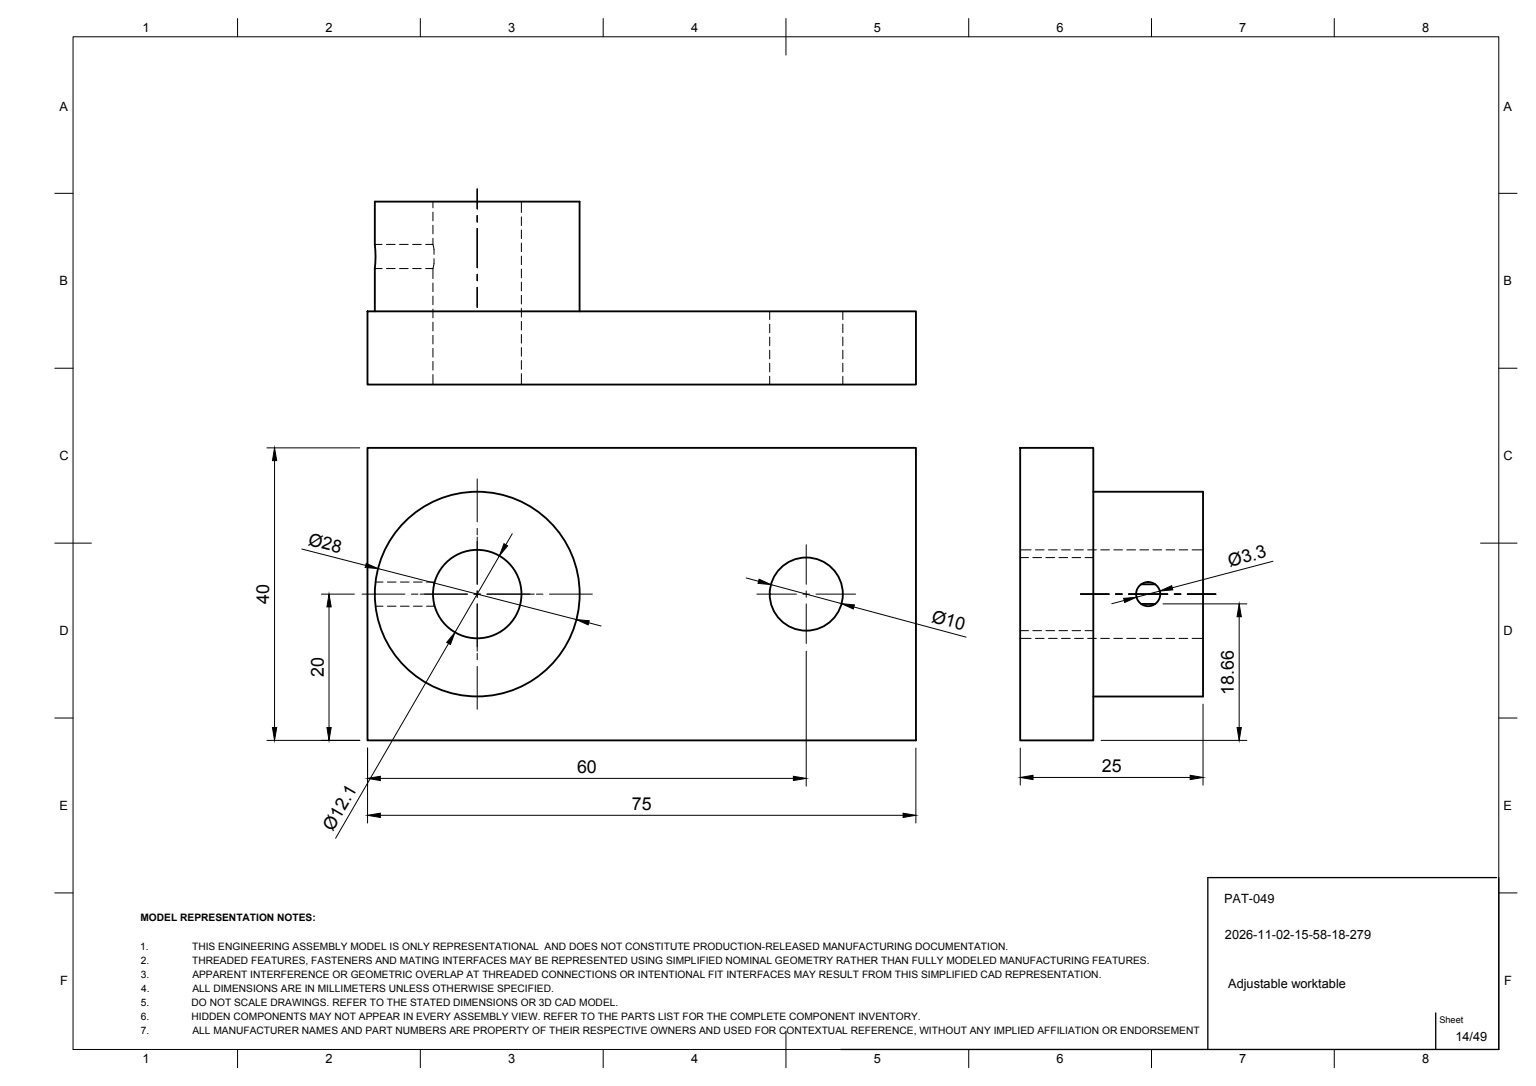
ISO-10303-21;
HEADER;
/* Generated by software containing ST-Developer
 * from STEP Tools, Inc. (www.steptools.com) 
 */

FILE_DESCRIPTION(
/* description */ ('Hand drill press frame (manual)'),
/* implementation_level */ '2;1');

FILE_NAME(
/* name */ 'Adjustable worktable.step',
/* time_stamp */ '2026-10-28T03:25:28-07:00',
/* author */ (''),
/* organization */ (''),
/* preprocessor_version */ 'ST-DEVELOPER v20.2',
/* originating_system */ 'Autodesk Translation Framework v15.17.0.0',
/* authorisation */ '');

FILE_SCHEMA (('AUTOMOTIVE_DESIGN { 1 0 10303 214 3 1 1 }'));
ENDSEC;

DATA;
#10=MECHANICAL_DESIGN_GEOMETRIC_PRESENTATION_REPRESENTATION('',(#628),#33299);
#501=B_SPLINE_CURVE_WITH_KNOTS('',3,(#18696,#18697,#18698,#18699,#18700,
#18701,#18702,#18703,#18704,#18705,#18706,#18707,#18708,#18709),
 .UNSPECIFIED.,.F.,.F.,(4,2,2,2,2,2,4),(0.598759573717651,0.624973342427791,
0.687463163426144,0.749952984424497,0.812442805422849,0.874932626421202,
0.901146395131343),.UNSPECIFIED.);
#502=B_SPLINE_CURVE_WITH_KNOTS('',3,(#18713,#18714,#18715,#18716,#18717,
#18718,#18719,#18720),.UNSPECIFIED.,.F.,.F.,(4,2,2,4),(0.249984328141499,
0.312474149139851,0.374963970138204,0.401177738848344),.UNSPECIFIED.);
#503=B_SPLINE_CURVE_WITH_KNOTS('',3,(#18724,#18725,#18726,#18727,#18728,
#18729,#18730,#18731,#18732,#18733,#18734,#18735,#18736,#18737,#18738,#18739,
#18740,#18741,#18742,#18743,#18744,#18745,#18746,#18747,#18748,#18749),
 .UNSPECIFIED.,.F.,.F.,(4,2,2,2,2,2,2,2,2,2,2,2,4),(0.,0.0622156192199746,
0.124431238439949,0.186646447577113,0.248861656714278,0.311076865851442,
0.373292074988606,0.43550769420858,0.497723313428555,0.55993893264853,0.622154551868504,
0.684369761005668,0.746584970142833),.UNSPECIFIED.);
#504=B_SPLINE_CURVE_WITH_KNOTS('',3,(#18750,#18751,#18752,#18753,#18754,
#18755,#18756,#18757,#18758,#18759),.UNSPECIFIED.,.F.,.F.,(4,2,2,2,4),(0.746584970142833,
0.808800179279997,0.871015388417161,0.933231007637136,0.99544662685711),
 .UNSPECIFIED.);
#505=B_SPLINE_CURVE_WITH_KNOTS('',3,(#18760,#18761,#18762,#18763,#18764,
#18765,#18766,#18767),.UNSPECIFIED.,.F.,.F.,(4,2,2,4),(0.0987909174346536,
0.125004686144794,0.187494507143146,0.249984328141499),.UNSPECIFIED.);
#538=SHAPE_REPRESENTATION_RELATIONSHIP('SRR','None',#33497,#583);
#583=ADVANCED_BREP_SHAPE_REPRESENTATION('',(#680),#33259);
#628=STYLED_ITEM('',(#33807),#680);
#680=MANIFOLD_SOLID_BREP('Body1',#12646);
#757=FACE_BOUND('',#2194,.T.);
#758=FACE_BOUND('',#2195,.T.);
#759=FACE_BOUND('',#2199,.T.);
#760=FACE_BOUND('',#2200,.T.);
#761=FACE_BOUND('',#2206,.T.);
#762=FACE_BOUND('',#2208,.T.);
#763=FACE_BOUND('',#2210,.T.);
#974=PLANE('',#13410);
#975=PLANE('',#13411);
#976=PLANE('',#13412);
#977=PLANE('',#13415);
#978=PLANE('',#13416);
#979=PLANE('',#13417);
#980=PLANE('',#13420);
#981=PLANE('',#13424);
#982=PLANE('',#13430);
#1465=FACE_OUTER_BOUND('',#2191,.T.);
#1466=FACE_OUTER_BOUND('',#2192,.T.);
#1467=FACE_OUTER_BOUND('',#2193,.T.);
#1468=FACE_OUTER_BOUND('',#2196,.T.);
#1469=FACE_OUTER_BOUND('',#2197,.T.);
#1470=FACE_OUTER_BOUND('',#2198,.T.);
#1471=FACE_OUTER_BOUND('',#2201,.T.);
#1472=FACE_OUTER_BOUND('',#2202,.T.);
#1473=FACE_OUTER_BOUND('',#2203,.T.);
#1474=FACE_OUTER_BOUND('',#2204,.T.);
#1475=FACE_OUTER_BOUND('',#2205,.T.);
#1476=FACE_OUTER_BOUND('',#2207,.T.);
#1477=FACE_OUTER_BOUND('',#2209,.T.);
#2191=EDGE_LOOP('',(#9027,#9028,#9029,#9030));
#2192=EDGE_LOOP('',(#9031,#9032,#9033,#9034));
#2193=EDGE_LOOP('',(#9035,#9036,#9037,#9038));
#2194=EDGE_LOOP('',(#9039));
#2195=EDGE_LOOP('',(#9040));
#2196=EDGE_LOOP('',(#9041,#9042,#9043,#9044));
#2197=EDGE_LOOP('',(#9045,#9046,#9047,#9048));
#2198=EDGE_LOOP('',(#9049,#9050,#9051,#9052));
#2199=EDGE_LOOP('',(#9053));
#2200=EDGE_LOOP('',(#9054));
#2201=EDGE_LOOP('',(#9055,#9056));
#2202=EDGE_LOOP('',(#9057,#9058,#9059,#9060,#9061,#9062,#9063,#9064,#9065));
#2203=EDGE_LOOP('',(#9066,#9067));
#2204=EDGE_LOOP('',(#9068,#9069,#9070,#9071));
#2205=EDGE_LOOP('',(#9072,#9073,#9074,#9075));
#2206=EDGE_LOOP('',(#9076,#9077,#9078,#9079,#9080));
#2207=EDGE_LOOP('',(#9081,#9082,#9083,#9084));
#2208=EDGE_LOOP('',(#9085,#9086));
#2209=EDGE_LOOP('',(#9087));
#2210=EDGE_LOOP('',(#9088));
#3093=LINE('',#18658,#4258);
#3094=LINE('',#18660,#4259);
#3095=LINE('',#18662,#4260);
#3096=LINE('',#18663,#4261);
#3097=LINE('',#18666,#4262);
#3098=LINE('',#18668,#4263);
#3099=LINE('',#18669,#4264);
#3100=LINE('',#18672,#4265);
#3101=LINE('',#18673,#4266);
#3102=LINE('',#18680,#4267);
#3103=LINE('',#18681,#4268);
#3104=LINE('',#18683,#4269);
#3105=LINE('',#18692,#4270);
#3106=LINE('',#18722,#4271);
#3107=LINE('',#18769,#4272);
#3108=LINE('',#18771,#4273);
#3109=LINE('',#18775,#4274);
#3110=LINE('',#18778,#4275);
#4258=VECTOR('',#15022,1.);
#4259=VECTOR('',#15023,1.);
#4260=VECTOR('',#15024,1.);
#4261=VECTOR('',#15025,1.);
#4262=VECTOR('',#15028,1.);
#4263=VECTOR('',#15029,1.);
#4264=VECTOR('',#15030,1.);
#4265=VECTOR('',#15033,1.);
#4266=VECTOR('',#15034,1.);
#4267=VECTOR('',#15041,1.);
#4268=VECTOR('',#15042,1.);
#4269=VECTOR('',#15045,1.);
#4270=VECTOR('',#15054,1.);
#4271=VECTOR('',#15061,0.165);
#4272=VECTOR('',#15064,1.);
#4273=VECTOR('',#15067,0.5);
#4274=VECTOR('',#15072,0.605);
#4275=VECTOR('',#15075,1.4);
#5298=CIRCLE('',#13413,0.5);
#5299=CIRCLE('',#13414,1.4);
#5300=CIRCLE('',#13418,0.605);
#5301=CIRCLE('',#13419,0.5);
#5302=CIRCLE('',#13421,0.165);
#5303=CIRCLE('',#13423,0.165);
#5304=CIRCLE('',#13427,0.605);
#5305=CIRCLE('',#13429,1.4);
#5815=VERTEX_POINT('',#18656);
#5816=VERTEX_POINT('',#18657);
#5817=VERTEX_POINT('',#18659);
#5818=VERTEX_POINT('',#18661);
#5819=VERTEX_POINT('',#18665);
#5820=VERTEX_POINT('',#18667);
#5821=VERTEX_POINT('',#18671);
#5822=VERTEX_POINT('',#18674);
#5823=VERTEX_POINT('',#18676);
#5824=VERTEX_POINT('',#18679);
#5825=VERTEX_POINT('',#18685);
#5826=VERTEX_POINT('',#18687);
#5827=VERTEX_POINT('',#18690);
#5828=VERTEX_POINT('',#18691);
#5829=VERTEX_POINT('',#18695);
#5830=VERTEX_POINT('',#18710);
#5831=VERTEX_POINT('',#18712);
#5832=VERTEX_POINT('',#18721);
#5833=VERTEX_POINT('',#18723);
#5834=VERTEX_POINT('',#18773);
#5835=VERTEX_POINT('',#18777);
#7042=EDGE_CURVE('',#5815,#5816,#3093,.T.);
#7043=EDGE_CURVE('',#5817,#5815,#3094,.T.);
#7044=EDGE_CURVE('',#5818,#5817,#3095,.T.);
#7045=EDGE_CURVE('',#5816,#5818,#3096,.T.);
#7046=EDGE_CURVE('',#5819,#5818,#3097,.T.);
#7047=EDGE_CURVE('',#5819,#5820,#3098,.T.);
#7048=EDGE_CURVE('',#5816,#5820,#3099,.T.);
#7049=EDGE_CURVE('',#5821,#5817,#3100,.T.);
#7050=EDGE_CURVE('',#5821,#5819,#3101,.T.);
#7051=EDGE_CURVE('',#5822,#5822,#5298,.T.);
#7052=EDGE_CURVE('',#5823,#5823,#5299,.T.);
#7053=EDGE_CURVE('',#5820,#5824,#3102,.T.);
#7054=EDGE_CURVE('',#5824,#5821,#3103,.T.);
#7055=EDGE_CURVE('',#5824,#5815,#3104,.T.);
#7056=EDGE_CURVE('',#5825,#5825,#5300,.T.);
#7057=EDGE_CURVE('',#5826,#5826,#5301,.T.);
#7058=EDGE_CURVE('',#5827,#5828,#3105,.T.);
#7059=EDGE_CURVE('',#5827,#5828,#5302,.T.);
#7060=EDGE_CURVE('',#5829,#5827,#501,.T.);
#7061=EDGE_CURVE('',#5830,#5829,#5303,.T.);
#7062=EDGE_CURVE('',#5831,#5830,#502,.T.);
#7063=EDGE_CURVE('',#5831,#5832,#3106,.T.);
#7064=EDGE_CURVE('',#5833,#5832,#503,.T.);
#7065=EDGE_CURVE('',#5832,#5833,#504,.T.);
#7066=EDGE_CURVE('',#5828,#5831,#505,.T.);
#7067=EDGE_CURVE('',#5830,#5829,#3107,.T.);
#7068=EDGE_CURVE('',#5822,#5826,#3108,.T.);
#7069=EDGE_CURVE('',#5834,#5834,#5304,.T.);
#7070=EDGE_CURVE('',#5834,#5825,#3109,.T.);
#7071=EDGE_CURVE('',#5823,#5835,#3110,.T.);
#7072=EDGE_CURVE('',#5835,#5835,#5305,.T.);
#9027=ORIENTED_EDGE('',*,*,#7042,.F.);
#9028=ORIENTED_EDGE('',*,*,#7043,.F.);
#9029=ORIENTED_EDGE('',*,*,#7044,.F.);
#9030=ORIENTED_EDGE('',*,*,#7045,.F.);
#9031=ORIENTED_EDGE('',*,*,#7045,.T.);
#9032=ORIENTED_EDGE('',*,*,#7046,.F.);
#9033=ORIENTED_EDGE('',*,*,#7047,.T.);
#9034=ORIENTED_EDGE('',*,*,#7048,.F.);
#9035=ORIENTED_EDGE('',*,*,#7044,.T.);
#9036=ORIENTED_EDGE('',*,*,#7049,.F.);
#9037=ORIENTED_EDGE('',*,*,#7050,.T.);
#9038=ORIENTED_EDGE('',*,*,#7046,.T.);
#9039=ORIENTED_EDGE('',*,*,#7051,.T.);
#9040=ORIENTED_EDGE('',*,*,#7052,.T.);
#9041=ORIENTED_EDGE('',*,*,#7053,.F.);
#9042=ORIENTED_EDGE('',*,*,#7047,.F.);
#9043=ORIENTED_EDGE('',*,*,#7050,.F.);
#9044=ORIENTED_EDGE('',*,*,#7054,.F.);
#9045=ORIENTED_EDGE('',*,*,#7043,.T.);
#9046=ORIENTED_EDGE('',*,*,#7055,.F.);
#9047=ORIENTED_EDGE('',*,*,#7054,.T.);
#9048=ORIENTED_EDGE('',*,*,#7049,.T.);
#9049=ORIENTED_EDGE('',*,*,#7042,.T.);
#9050=ORIENTED_EDGE('',*,*,#7048,.T.);
#9051=ORIENTED_EDGE('',*,*,#7053,.T.);
#9052=ORIENTED_EDGE('',*,*,#7055,.T.);
#9053=ORIENTED_EDGE('',*,*,#7056,.T.);
#9054=ORIENTED_EDGE('',*,*,#7057,.T.);
#9055=ORIENTED_EDGE('',*,*,#7058,.F.);
#9056=ORIENTED_EDGE('',*,*,#7059,.T.);
#9057=ORIENTED_EDGE('',*,*,#7060,.F.);
#9058=ORIENTED_EDGE('',*,*,#7061,.F.);
#9059=ORIENTED_EDGE('',*,*,#7062,.F.);
#9060=ORIENTED_EDGE('',*,*,#7063,.T.);
#9061=ORIENTED_EDGE('',*,*,#7064,.F.);
#9062=ORIENTED_EDGE('',*,*,#7065,.F.);
#9063=ORIENTED_EDGE('',*,*,#7063,.F.);
#9064=ORIENTED_EDGE('',*,*,#7066,.F.);
#9065=ORIENTED_EDGE('',*,*,#7059,.F.);
#9066=ORIENTED_EDGE('',*,*,#7067,.F.);
#9067=ORIENTED_EDGE('',*,*,#7061,.T.);
#9068=ORIENTED_EDGE('',*,*,#7051,.F.);
#9069=ORIENTED_EDGE('',*,*,#7068,.T.);
#9070=ORIENTED_EDGE('',*,*,#7057,.F.);
#9071=ORIENTED_EDGE('',*,*,#7068,.F.);
#9072=ORIENTED_EDGE('',*,*,#7069,.F.);
#9073=ORIENTED_EDGE('',*,*,#7070,.T.);
#9074=ORIENTED_EDGE('',*,*,#7056,.F.);
#9075=ORIENTED_EDGE('',*,*,#7070,.F.);
#9076=ORIENTED_EDGE('',*,*,#7066,.T.);
#9077=ORIENTED_EDGE('',*,*,#7062,.T.);
#9078=ORIENTED_EDGE('',*,*,#7067,.T.);
#9079=ORIENTED_EDGE('',*,*,#7060,.T.);
#9080=ORIENTED_EDGE('',*,*,#7058,.T.);
#9081=ORIENTED_EDGE('',*,*,#7052,.F.);
#9082=ORIENTED_EDGE('',*,*,#7071,.T.);
#9083=ORIENTED_EDGE('',*,*,#7072,.T.);
#9084=ORIENTED_EDGE('',*,*,#7071,.F.);
#9085=ORIENTED_EDGE('',*,*,#7064,.T.);
#9086=ORIENTED_EDGE('',*,*,#7065,.T.);
#9087=ORIENTED_EDGE('',*,*,#7072,.F.);
#9088=ORIENTED_EDGE('',*,*,#7069,.T.);
#11824=CYLINDRICAL_SURFACE('',#13422,0.165);
#11825=CYLINDRICAL_SURFACE('',#13425,0.5);
#11826=CYLINDRICAL_SURFACE('',#13426,0.605);
#11827=CYLINDRICAL_SURFACE('',#13428,1.4);
#12074=ADVANCED_FACE('',(#1465),#974,.F.);
#12075=ADVANCED_FACE('',(#1466),#975,.F.);
#12076=ADVANCED_FACE('',(#1467,#757,#758),#976,.F.);
#12077=ADVANCED_FACE('',(#1468),#977,.F.);
#12078=ADVANCED_FACE('',(#1469),#978,.T.);
#12079=ADVANCED_FACE('',(#1470,#759,#760),#979,.T.);
#12080=ADVANCED_FACE('',(#1471),#980,.T.);
#12081=ADVANCED_FACE('',(#1472),#11824,.F.);
#12082=ADVANCED_FACE('',(#1473),#981,.T.);
#12083=ADVANCED_FACE('',(#1474),#11825,.F.);
#12084=ADVANCED_FACE('',(#1475,#761),#11826,.F.);
#12085=ADVANCED_FACE('',(#1476,#762),#11827,.T.);
#12086=ADVANCED_FACE('',(#1477,#763),#982,.F.);
#12646=CLOSED_SHELL('',(#12074,#12075,#12076,#12077,#12078,#12079,#12080,
#12081,#12082,#12083,#12084,#12085,#12086));
#13409=AXIS2_PLACEMENT_3D('',#18654,#15018,#15019);
#13410=AXIS2_PLACEMENT_3D('',#18655,#15020,#15021);
#13411=AXIS2_PLACEMENT_3D('',#18664,#15026,#15027);
#13412=AXIS2_PLACEMENT_3D('',#18670,#15031,#15032);
#13413=AXIS2_PLACEMENT_3D('',#18675,#15035,#15036);
#13414=AXIS2_PLACEMENT_3D('',#18677,#15037,#15038);
#13415=AXIS2_PLACEMENT_3D('',#18678,#15039,#15040);
#13416=AXIS2_PLACEMENT_3D('',#18682,#15043,#15044);
#13417=AXIS2_PLACEMENT_3D('',#18684,#15046,#15047);
#13418=AXIS2_PLACEMENT_3D('',#18686,#15048,#15049);
#13419=AXIS2_PLACEMENT_3D('',#18688,#15050,#15051);
#13420=AXIS2_PLACEMENT_3D('',#18689,#15052,#15053);
#13421=AXIS2_PLACEMENT_3D('',#18693,#15055,#15056);
#13422=AXIS2_PLACEMENT_3D('',#18694,#15057,#15058);
#13423=AXIS2_PLACEMENT_3D('',#18711,#15059,#15060);
#13424=AXIS2_PLACEMENT_3D('',#18768,#15062,#15063);
#13425=AXIS2_PLACEMENT_3D('',#18770,#15065,#15066);
#13426=AXIS2_PLACEMENT_3D('',#18772,#15068,#15069);
#13427=AXIS2_PLACEMENT_3D('',#18774,#15070,#15071);
#13428=AXIS2_PLACEMENT_3D('',#18776,#15073,#15074);
#13429=AXIS2_PLACEMENT_3D('',#18779,#15076,#15077);
#13430=AXIS2_PLACEMENT_3D('',#18780,#15078,#15079);
#15018=DIRECTION('axis',(0.,0.,1.));
#15019=DIRECTION('refdir',(1.,0.,0.));
#15020=DIRECTION('center_axis',(0.,-1.,0.));
#15021=DIRECTION('ref_axis',(1.,0.,0.));
#15022=DIRECTION('',(-1.,0.,0.));
#15023=DIRECTION('',(0.,0.,1.));
#15024=DIRECTION('',(1.,0.,0.));
#15025=DIRECTION('',(0.,0.,-1.));
#15026=DIRECTION('center_axis',(1.,0.,0.));
#15027=DIRECTION('ref_axis',(0.,1.,0.));
#15028=DIRECTION('',(0.,1.,0.));
#15029=DIRECTION('',(0.,0.,1.));
#15030=DIRECTION('',(0.,-1.,0.));
#15031=DIRECTION('center_axis',(0.,0.,1.));
#15032=DIRECTION('ref_axis',(1.,0.,0.));
#15033=DIRECTION('',(0.,1.,0.));
#15034=DIRECTION('',(-1.,0.,0.));
#15035=DIRECTION('center_axis',(0.,0.,1.));
#15036=DIRECTION('ref_axis',(1.,0.,0.));
#15037=DIRECTION('center_axis',(0.,0.,1.));
#15038=DIRECTION('ref_axis',(1.,0.,0.));
#15039=DIRECTION('center_axis',(0.,1.,0.));
#15040=DIRECTION('ref_axis',(-1.,0.,0.));
#15041=DIRECTION('',(1.,0.,0.));
#15042=DIRECTION('',(0.,0.,-1.));
#15043=DIRECTION('center_axis',(1.,0.,0.));
#15044=DIRECTION('ref_axis',(0.,1.,0.));
#15045=DIRECTION('',(0.,1.,0.));
#15046=DIRECTION('center_axis',(0.,0.,1.));
#15047=DIRECTION('ref_axis',(1.,0.,0.));
#15048=DIRECTION('center_axis',(0.,0.,-1.));
#15049=DIRECTION('ref_axis',(1.,0.,0.));
#15050=DIRECTION('center_axis',(0.,0.,-1.));
#15051=DIRECTION('ref_axis',(1.,0.,0.));
#15052=DIRECTION('center_axis',(1.,0.,0.));
#15053=DIRECTION('ref_axis',(0.,0.,-1.));
#15054=DIRECTION('',(0.,0.,1.));
#15055=DIRECTION('center_axis',(1.,0.,0.));
#15056=DIRECTION('ref_axis',(0.,0.,-1.));
#15057=DIRECTION('center_axis',(1.,0.,0.));
#15058=DIRECTION('ref_axis',(0.,0.,-1.));
#15059=DIRECTION('center_axis',(1.,0.,0.));
#15060=DIRECTION('ref_axis',(0.,0.,-1.));
#15061=DIRECTION('',(1.,0.,0.));
#15062=DIRECTION('center_axis',(1.,0.,0.));
#15063=DIRECTION('ref_axis',(0.,0.,-1.));
#15064=DIRECTION('',(0.,0.,-1.));
#15065=DIRECTION('center_axis',(0.,0.,1.));
#15066=DIRECTION('ref_axis',(1.,0.,0.));
#15067=DIRECTION('',(0.,0.,1.));
#15068=DIRECTION('center_axis',(0.,0.,1.));
#15069=DIRECTION('ref_axis',(1.,0.,0.));
#15070=DIRECTION('center_axis',(0.,0.,1.));
#15071=DIRECTION('ref_axis',(1.,0.,0.));
#15072=DIRECTION('',(0.,0.,1.));
#15073=DIRECTION('center_axis',(0.,0.,1.));
#15074=DIRECTION('ref_axis',(1.,0.,0.));
#15075=DIRECTION('',(0.,0.,-1.));
#15076=DIRECTION('center_axis',(0.,0.,1.));
#15077=DIRECTION('ref_axis',(1.,0.,0.));
#15078=DIRECTION('center_axis',(0.,0.,1.));
#15079=DIRECTION('ref_axis',(1.,0.,0.));
#18654=CARTESIAN_POINT('',(0.,0.,0.));
#18655=CARTESIAN_POINT('Origin',(-0.5,2.,4.4));
#18656=CARTESIAN_POINT('',(7.,2.,5.5));
#18657=CARTESIAN_POINT('',(-0.5,2.,5.5));
#18658=CARTESIAN_POINT('',(0.5,2.,5.5));
#18659=CARTESIAN_POINT('',(7.,2.,4.5));
#18660=CARTESIAN_POINT('',(7.,2.,4.45));
#18661=CARTESIAN_POINT('',(-0.5,2.,4.5));
#18662=CARTESIAN_POINT('',(0.5,2.,4.5));
#18663=CARTESIAN_POINT('',(-0.5,2.,4.4));
#18664=CARTESIAN_POINT('Origin',(-0.5,-4.1,4.4));
#18665=CARTESIAN_POINT('',(-0.5,-2.,4.5));
#18666=CARTESIAN_POINT('',(-0.5,-2.05,4.5));
#18667=CARTESIAN_POINT('',(-0.5,-2.,5.5));
#18668=CARTESIAN_POINT('',(-0.5,-2.,4.4));
#18669=CARTESIAN_POINT('',(-0.5,-2.05,5.5));
#18670=CARTESIAN_POINT('Origin',(1.5,0.,4.5));
#18671=CARTESIAN_POINT('',(7.,-2.,4.5));
#18672=CARTESIAN_POINT('',(7.,-4.,4.5));
#18673=CARTESIAN_POINT('',(4.3,-2.,4.5));
#18674=CARTESIAN_POINT('',(0.5,-6.12323399573677E-17,4.5));
#18675=CARTESIAN_POINT('Origin',(1.,0.,4.5));
#18676=CARTESIAN_POINT('',(4.1,-1.71450551880629E-16,4.5));
#18677=CARTESIAN_POINT('Origin',(5.5,0.,4.5));
#18678=CARTESIAN_POINT('Origin',(7.1,-2.,4.4));
#18679=CARTESIAN_POINT('',(7.,-2.,5.5));
#18680=CARTESIAN_POINT('',(4.3,-2.,5.5));
#18681=CARTESIAN_POINT('',(7.,-2.,4.45));
#18682=CARTESIAN_POINT('Origin',(7.,-4.,4.5));
#18683=CARTESIAN_POINT('',(7.,-4.,5.5));
#18684=CARTESIAN_POINT('Origin',(1.5,0.,5.5));
#18685=CARTESIAN_POINT('',(4.895,7.40911313484149E-17,5.5));
#18686=CARTESIAN_POINT('Origin',(5.5,0.,5.5));
#18687=CARTESIAN_POINT('',(0.5,6.12323399573677E-17,5.5));
#18688=CARTESIAN_POINT('Origin',(1.,0.,5.5));
#18689=CARTESIAN_POINT('Origin',(6.09,0.,3.75));
#18690=CARTESIAN_POINT('',(6.09,0.133884278389961,3.65356349239007));
#18691=CARTESIAN_POINT('',(6.09,0.133884278389961,3.84643650760993));
#18692=CARTESIAN_POINT('',(6.09,0.133884278389961,2.9));
#18693=CARTESIAN_POINT('Origin',(6.09,0.,3.75));
#18694=CARTESIAN_POINT('Origin',(6.09,0.,3.75));
#18695=CARTESIAN_POINT('',(6.09,-0.133884278389961,3.65356349239007));
#18696=CARTESIAN_POINT('Ctrl Pts',(6.09,-0.133884278389961,3.65356349239007));
#18697=CARTESIAN_POINT('Ctrl Pts',(6.09119840340611,-0.128603165341395,
3.64623164237677));
#18698=CARTESIAN_POINT('Ctrl Pts',(6.09244064128815,-0.122792448979944,
3.63944721118838));
#18699=CARTESIAN_POINT('Ctrl Pts',(6.09651064111414,-0.10208383195986,3.6187385941683));
#18700=CARTESIAN_POINT('Ctrl Pts',(6.09954409498317,-0.0836002135946606,
3.6060565239921));
#18701=CARTESIAN_POINT('Ctrl Pts',(6.10381707438298,-0.0429774150042654,
3.5891843843662));
#18702=CARTESIAN_POINT('Ctrl Pts',(6.105,-0.0208299403327843,3.585));
#18703=CARTESIAN_POINT('Ctrl Pts',(6.105,0.0208299403327842,3.585));
#18704=CARTESIAN_POINT('Ctrl Pts',(6.10381707438298,0.0429774150042653,
3.5891843843662));
#18705=CARTESIAN_POINT('Ctrl Pts',(6.09954409498317,0.0836002135946605,
3.6060565239921));
#18706=CARTESIAN_POINT('Ctrl Pts',(6.09651064111414,0.10208383195986,3.6187385941683));
#18707=CARTESIAN_POINT('Ctrl Pts',(6.09244064128815,0.122792448979944,3.63944721118838));
#18708=CARTESIAN_POINT('Ctrl Pts',(6.09119840340611,0.128603165341395,3.64623164237677));
#18709=CARTESIAN_POINT('Ctrl Pts',(6.09,0.133884278389961,3.65356349239007));
#18710=CARTESIAN_POINT('',(6.09,-0.133884278389961,3.84643650760993));
#18711=CARTESIAN_POINT('Origin',(6.09,0.,3.75));
#18712=CARTESIAN_POINT('',(6.105,-4.82672525644554E-17,3.915));
#18713=CARTESIAN_POINT('Ctrl Pts',(6.105,-6.93889390390723E-17,3.915));
#18714=CARTESIAN_POINT('Ctrl Pts',(6.105,-0.0208299403327843,3.915));
#18715=CARTESIAN_POINT('Ctrl Pts',(6.10381707438298,-0.0429774150042653,
3.9108156156338));
#18716=CARTESIAN_POINT('Ctrl Pts',(6.09954409498317,-0.0836002135946605,
3.8939434760079));
#18717=CARTESIAN_POINT('Ctrl Pts',(6.09651064111414,-0.10208383195986,3.8812614058317));
#18718=CARTESIAN_POINT('Ctrl Pts',(6.09244064128815,-0.122792448979944,
3.86055278881162));
#18719=CARTESIAN_POINT('Ctrl Pts',(6.09119840340611,-0.128603165341395,
3.85376835762323));
#18720=CARTESIAN_POINT('Ctrl Pts',(6.09,-0.133884278389961,3.84643650760993));
#18721=CARTESIAN_POINT('',(6.9,-2.02066721859313E-17,3.915));
#18722=CARTESIAN_POINT('',(6.09,-2.02066721859313E-17,3.915));
#18723=CARTESIAN_POINT('',(6.8902427845524,0.165,3.75));
#18724=CARTESIAN_POINT('Ctrl Pts',(6.8902427845524,0.165,3.75));
#18725=CARTESIAN_POINT('Ctrl Pts',(6.8902427845524,0.165,3.72926146026001));
#18726=CARTESIAN_POINT('Ctrl Pts',(6.89075468722975,0.160851447474559,3.70715388604164));
#18727=CARTESIAN_POINT('Ctrl Pts',(6.89259968365095,0.144006627864301,3.6665070705051));
#18728=CARTESIAN_POINT('Ctrl Pts',(6.89390570229761,0.131311408395222,3.64796617060366));
#18729=CARTESIAN_POINT('Ctrl Pts',(6.89635413416378,0.102033925885227,3.61868868809367));
#18730=CARTESIAN_POINT('Ctrl Pts',(6.89765618378145,0.0834929839417279,
3.60599339308932));
#18731=CARTESIAN_POINT('Ctrl Pts',(6.89949208802221,0.0428460264460559,
3.58914851786885));
#18732=CARTESIAN_POINT('Ctrl Pts',(6.9,0.0207384030457214,3.585));
#18733=CARTESIAN_POINT('Ctrl Pts',(6.9,-0.0207384030457214,3.585));
#18734=CARTESIAN_POINT('Ctrl Pts',(6.89949208802221,-0.0428460264460559,
3.58914851786885));
#18735=CARTESIAN_POINT('Ctrl Pts',(6.89765618378145,-0.0834929839417279,
3.60599339308932));
#18736=CARTESIAN_POINT('Ctrl Pts',(6.89635413416378,-0.102033925885227,
3.61868868809367));
#18737=CARTESIAN_POINT('Ctrl Pts',(6.89390570229761,-0.131311408395222,
3.64796617060366));
#18738=CARTESIAN_POINT('Ctrl Pts',(6.89259968365095,-0.144006627864301,
3.6665070705051));
#18739=CARTESIAN_POINT('Ctrl Pts',(6.89075468722975,-0.160851447474559,
3.70715388604164));
#18740=CARTESIAN_POINT('Ctrl Pts',(6.8902427845524,-0.165,3.72926146026001));
#18741=CARTESIAN_POINT('Ctrl Pts',(6.8902427845524,-0.165,3.77073853973999));
#18742=CARTESIAN_POINT('Ctrl Pts',(6.89075468722975,-0.160851447474559,
3.79284611395836));
#18743=CARTESIAN_POINT('Ctrl Pts',(6.89259968365095,-0.144006627864301,
3.8334929294949));
#18744=CARTESIAN_POINT('Ctrl Pts',(6.89390570229761,-0.131311408395222,
3.85203382939634));
#18745=CARTESIAN_POINT('Ctrl Pts',(6.89635413416378,-0.102033925885227,
3.88131131190633));
#18746=CARTESIAN_POINT('Ctrl Pts',(6.89765618378145,-0.0834929839417278,
3.89400660691068));
#18747=CARTESIAN_POINT('Ctrl Pts',(6.89949208802221,-0.0428460264460559,
3.91085148213115));
#18748=CARTESIAN_POINT('Ctrl Pts',(6.9,-0.0207384030457214,3.915));
#18749=CARTESIAN_POINT('Ctrl Pts',(6.9,-7.63278329429795E-17,3.915));
#18750=CARTESIAN_POINT('Ctrl Pts',(6.9,-3.46944695195361E-17,3.915));
#18751=CARTESIAN_POINT('Ctrl Pts',(6.9,0.0207384030457214,3.915));
#18752=CARTESIAN_POINT('Ctrl Pts',(6.89949208802221,0.0428460264460559,
3.91085148213115));
#18753=CARTESIAN_POINT('Ctrl Pts',(6.89765618378145,0.0834929839417279,
3.89400660691068));
#18754=CARTESIAN_POINT('Ctrl Pts',(6.89635413416378,0.102033925885227,3.88131131190633));
#18755=CARTESIAN_POINT('Ctrl Pts',(6.89390570229761,0.131311408395222,3.85203382939634));
#18756=CARTESIAN_POINT('Ctrl Pts',(6.89259968365095,0.144006627864301,3.8334929294949));
#18757=CARTESIAN_POINT('Ctrl Pts',(6.89075468722975,0.160851447474559,3.79284611395836));
#18758=CARTESIAN_POINT('Ctrl Pts',(6.8902427845524,0.165,3.77073853973999));
#18759=CARTESIAN_POINT('Ctrl Pts',(6.8902427845524,0.165,3.75));
#18760=CARTESIAN_POINT('Ctrl Pts',(6.09,0.133884278389961,3.84643650760993));
#18761=CARTESIAN_POINT('Ctrl Pts',(6.09119840340611,0.128603165341395,3.85376835762323));
#18762=CARTESIAN_POINT('Ctrl Pts',(6.09244064128815,0.122792448979944,3.86055278881162));
#18763=CARTESIAN_POINT('Ctrl Pts',(6.09651064111414,0.10208383195986,3.8812614058317));
#18764=CARTESIAN_POINT('Ctrl Pts',(6.09954409498317,0.0836002135946605,
3.8939434760079));
#18765=CARTESIAN_POINT('Ctrl Pts',(6.10381707438298,0.0429774150042653,
3.9108156156338));
#18766=CARTESIAN_POINT('Ctrl Pts',(6.105,0.0208299403327843,3.915));
#18767=CARTESIAN_POINT('Ctrl Pts',(6.105,9.0205620750794E-17,3.915));
#18768=CARTESIAN_POINT('Origin',(6.09,0.,3.75));
#18769=CARTESIAN_POINT('',(6.09,-0.133884278389961,2.9));
#18770=CARTESIAN_POINT('Origin',(1.,0.,4.4));
#18771=CARTESIAN_POINT('',(0.5,-6.12323399573677E-17,4.4));
#18772=CARTESIAN_POINT('Origin',(5.5,0.,2.9));
#18773=CARTESIAN_POINT('',(4.895,-7.40911313484149E-17,3.));
#18774=CARTESIAN_POINT('Origin',(5.5,0.,3.));
#18775=CARTESIAN_POINT('',(4.895,-7.40911313484149E-17,2.9));
#18776=CARTESIAN_POINT('Origin',(5.5,0.,3.));
#18777=CARTESIAN_POINT('',(4.1,-1.71450551880629E-16,3.));
#18778=CARTESIAN_POINT('',(4.1,-1.71450551880629E-16,3.));
#18779=CARTESIAN_POINT('Origin',(5.5,0.,3.));
#18780=CARTESIAN_POINT('Origin',(5.5,0.,3.));
#33207=UNCERTAINTY_MEASURE_WITH_UNIT(LENGTH_MEASURE(0.001),#33300,
'DISTANCE_ACCURACY_VALUE',
'Maximum model space distance between geometric entities at asserted c
onnectivities');
#33247=UNCERTAINTY_MEASURE_WITH_UNIT(LENGTH_MEASURE(0.001),#33300,
'DISTANCE_ACCURACY_VALUE',
'Maximum model space distance between geometric entities at asserted c
onnectivities');
#33259=(
GEOMETRIC_REPRESENTATION_CONTEXT(3)
GLOBAL_UNCERTAINTY_ASSIGNED_CONTEXT((#33207))
GLOBAL_UNIT_ASSIGNED_CONTEXT((#33300,#33302,#33303))
REPRESENTATION_CONTEXT('','3D')
);
#33299=(
GEOMETRIC_REPRESENTATION_CONTEXT(3)
GLOBAL_UNCERTAINTY_ASSIGNED_CONTEXT((#33247))
GLOBAL_UNIT_ASSIGNED_CONTEXT((#33300,#33302,#33303))
REPRESENTATION_CONTEXT('','3D')
);
#33300=(
LENGTH_UNIT()
NAMED_UNIT(*)
SI_UNIT(.CENTI.,.METRE.)
);
#33302=(
NAMED_UNIT(*)
PLANE_ANGLE_UNIT()
SI_UNIT($,.RADIAN.)
);
#33303=(
NAMED_UNIT(*)
SI_UNIT($,.STERADIAN.)
SOLID_ANGLE_UNIT()
);
#33315=SHAPE_DEFINITION_REPRESENTATION(#33366,#33497);
#33366=PRODUCT_DEFINITION_SHAPE('',$,#33549);
#33497=SHAPE_REPRESENTATION('',(#13409),#33259);
#33537=PRODUCT_DEFINITION_CONTEXT('part definition',#33692,'design');
#33549=PRODUCT_DEFINITION('Adjustable worktable','Adjustable worktable',
#33600,#33537);
#33600=PRODUCT_DEFINITION_FORMATION('',$,#33705);
#33692=APPLICATION_CONTEXT(
'Core Data for Automotive Mechanical Design Process');
#33693=PRODUCT_CONTEXT('part definition',#33692,'mechanical');
#33705=PRODUCT('Adjustable worktable','Adjustable worktable',
'Adjustable worktable',(#33693));
#33801=COLOUR_RGB('Sky Blue',0.24,0.69,0.87);
#33802=FILL_AREA_STYLE_COLOUR('',#33801);
#33803=FILL_AREA_STYLE('',(#33802));
#33804=SURFACE_STYLE_FILL_AREA(#33803);
#33805=SURFACE_SIDE_STYLE('',(#33804));
#33806=SURFACE_STYLE_USAGE(.BOTH.,#33805);
#33807=PRESENTATION_STYLE_ASSIGNMENT((#33806));
ENDSEC;
END-ISO-10303-21;
